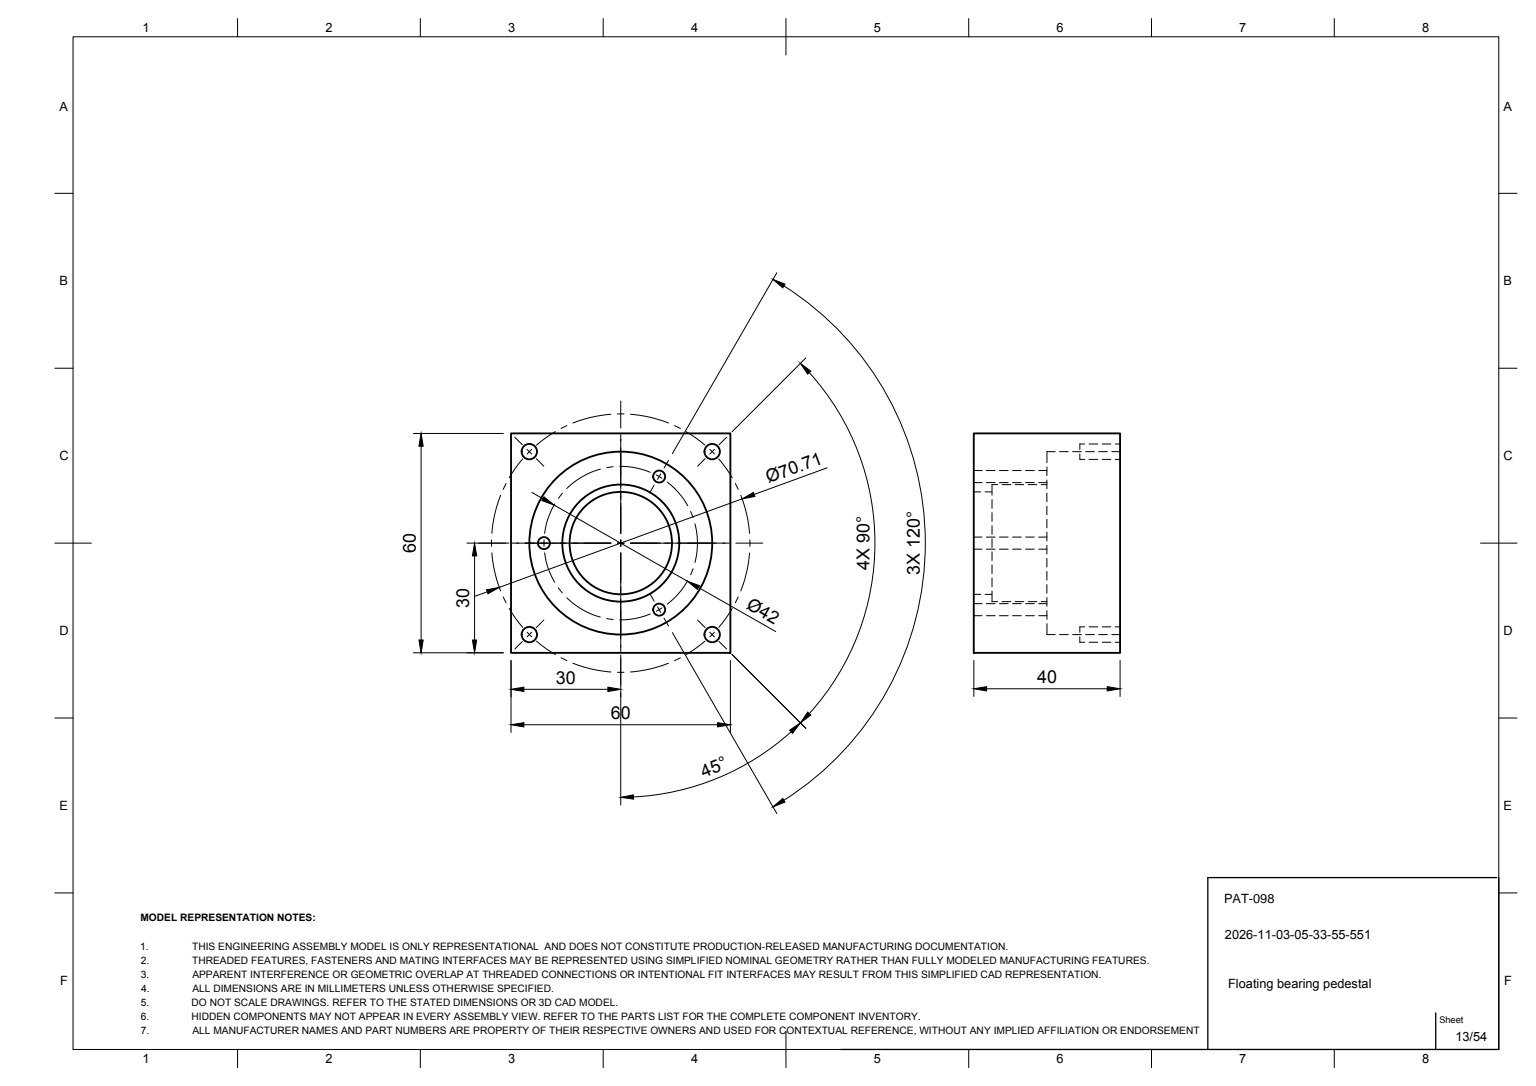
ISO-10303-21;
HEADER;
/* Generated by software containing ST-Developer
 * from STEP Tools, Inc. (www.steptools.com) 
 */

FILE_DESCRIPTION(
/* description */ ('Spring compression tester'),
/* implementation_level */ '2;1');

FILE_NAME(
/* name */ 'Floating bearing pedestal.step',
/* time_stamp */ '2026-10-28T03:24:11-07:00',
/* author */ (''),
/* organization */ (''),
/* preprocessor_version */ 'ST-DEVELOPER v20.2',
/* originating_system */ 'Autodesk Translation Framework v15.17.0.0',
/* authorisation */ '');

FILE_SCHEMA (('AUTOMOTIVE_DESIGN { 1 0 10303 214 3 1 1 }'));
ENDSEC;

DATA;
#10=MECHANICAL_DESIGN_GEOMETRIC_PRESENTATION_REPRESENTATION('',(#1114),#43521);
#994=SHAPE_REPRESENTATION_RELATIONSHIP('SRR','None',#43806,#1054);
#1054=ADVANCED_BREP_SHAPE_REPRESENTATION('',(#1189),#43466);
#1114=STYLED_ITEM('',(#44202),#1189);
#1189=MANIFOLD_SOLID_BREP('Body1',#18551);
#1345=FACE_BOUND('',#3478,.T.);
#1346=FACE_BOUND('',#3482,.T.);
#1347=FACE_BOUND('',#3483,.T.);
#1348=FACE_BOUND('',#3484,.T.);
#1349=FACE_BOUND('',#3485,.T.);
#1350=FACE_BOUND('',#3491,.T.);
#1351=FACE_BOUND('',#3492,.T.);
#1352=FACE_BOUND('',#3493,.T.);
#1353=FACE_BOUND('',#3494,.T.);
#1354=FACE_BOUND('',#3496,.T.);
#1355=FACE_BOUND('',#3497,.T.);
#1356=FACE_BOUND('',#3498,.T.);
#1357=FACE_BOUND('',#3499,.T.);
#1358=FACE_BOUND('',#3500,.T.);
#1681=PLANE('',#19583);
#1682=PLANE('',#19587);
#1683=PLANE('',#19591);
#1684=PLANE('',#19595);
#1685=PLANE('',#19599);
#1686=PLANE('',#19606);
#1687=PLANE('',#19607);
#1688=PLANE('',#19608);
#1689=PLANE('',#19609);
#1690=PLANE('',#19610);
#1691=PLANE('',#19611);
#1692=PLANE('',#19612);
#2320=FACE_OUTER_BOUND('',#3465,.T.);
#2321=FACE_OUTER_BOUND('',#3466,.T.);
#2322=FACE_OUTER_BOUND('',#3467,.T.);
#2323=FACE_OUTER_BOUND('',#3468,.T.);
#2324=FACE_OUTER_BOUND('',#3469,.T.);
#2325=FACE_OUTER_BOUND('',#3470,.T.);
#2326=FACE_OUTER_BOUND('',#3471,.T.);
#2327=FACE_OUTER_BOUND('',#3472,.T.);
#2328=FACE_OUTER_BOUND('',#3473,.T.);
#2329=FACE_OUTER_BOUND('',#3474,.T.);
#2330=FACE_OUTER_BOUND('',#3475,.T.);
#2331=FACE_OUTER_BOUND('',#3476,.T.);
#2332=FACE_OUTER_BOUND('',#3477,.T.);
#2333=FACE_OUTER_BOUND('',#3479,.T.);
#2334=FACE_OUTER_BOUND('',#3480,.T.);
#2335=FACE_OUTER_BOUND('',#3481,.T.);
#2336=FACE_OUTER_BOUND('',#3486,.T.);
#2337=FACE_OUTER_BOUND('',#3487,.T.);
#2338=FACE_OUTER_BOUND('',#3488,.T.);
#2339=FACE_OUTER_BOUND('',#3489,.T.);
#2340=FACE_OUTER_BOUND('',#3490,.T.);
#2341=FACE_OUTER_BOUND('',#3495,.T.);
#3465=EDGE_LOOP('',(#12925,#12926,#12927,#12928));
#3466=EDGE_LOOP('',(#12929,#12930,#12931,#12932));
#3467=EDGE_LOOP('',(#12933,#12934,#12935,#12936));
#3468=EDGE_LOOP('',(#12937,#12938,#12939,#12940));
#3469=EDGE_LOOP('',(#12941));
#3470=EDGE_LOOP('',(#12942,#12943,#12944,#12945));
#3471=EDGE_LOOP('',(#12946));
#3472=EDGE_LOOP('',(#12947,#12948,#12949,#12950));
#3473=EDGE_LOOP('',(#12951));
#3474=EDGE_LOOP('',(#12952,#12953,#12954,#12955));
#3475=EDGE_LOOP('',(#12956));
#3476=EDGE_LOOP('',(#12957,#12958,#12959,#12960));
#3477=EDGE_LOOP('',(#12961));
#3478=EDGE_LOOP('',(#12962));
#3479=EDGE_LOOP('',(#12963,#12964,#12965,#12966));
#3480=EDGE_LOOP('',(#12967,#12968,#12969,#12970));
#3481=EDGE_LOOP('',(#12971));
#3482=EDGE_LOOP('',(#12972));
#3483=EDGE_LOOP('',(#12973));
#3484=EDGE_LOOP('',(#12974));
#3485=EDGE_LOOP('',(#12975));
#3486=EDGE_LOOP('',(#12976,#12977,#12978,#12979));
#3487=EDGE_LOOP('',(#12980,#12981,#12982,#12983));
#3488=EDGE_LOOP('',(#12984,#12985,#12986,#12987));
#3489=EDGE_LOOP('',(#12988,#12989,#12990,#12991));
#3490=EDGE_LOOP('',(#12992,#12993,#12994,#12995));
#3491=EDGE_LOOP('',(#12996));
#3492=EDGE_LOOP('',(#12997));
#3493=EDGE_LOOP('',(#12998));
#3494=EDGE_LOOP('',(#12999));
#3495=EDGE_LOOP('',(#13000,#13001,#13002,#13003));
#3496=EDGE_LOOP('',(#13004));
#3497=EDGE_LOOP('',(#13005));
#3498=EDGE_LOOP('',(#13006));
#3499=EDGE_LOOP('',(#13007));
#3500=EDGE_LOOP('',(#13008));
#4836=LINE('',#27209,#6268);
#4837=LINE('',#27215,#6269);
#4838=LINE('',#27221,#6270);
#4839=LINE('',#27227,#6271);
#4840=LINE('',#27234,#6272);
#4841=LINE('',#27241,#6273);
#4842=LINE('',#27248,#6274);
#4843=LINE('',#27255,#6275);
#4844=LINE('',#27262,#6276);
#4845=LINE('',#27268,#6277);
#4846=LINE('',#27274,#6278);
#4847=LINE('',#27276,#6279);
#4848=LINE('',#27278,#6280);
#4849=LINE('',#27279,#6281);
#4850=LINE('',#27282,#6282);
#4851=LINE('',#27284,#6283);
#4852=LINE('',#27285,#6284);
#4853=LINE('',#27288,#6285);
#4854=LINE('',#27290,#6286);
#4855=LINE('',#27291,#6287);
#4856=LINE('',#27293,#6288);
#4857=LINE('',#27294,#6289);
#6268=VECTOR('',#22004,0.165);
#6269=VECTOR('',#22011,0.165);
#6270=VECTOR('',#22018,0.165);
#6271=VECTOR('',#22025,0.21);
#6272=VECTOR('',#22034,0.21);
#6273=VECTOR('',#22043,0.21);
#6274=VECTOR('',#22052,0.21);
#6275=VECTOR('',#22061,1.6);
#6276=VECTOR('',#22070,1.4);
#6277=VECTOR('',#22077,2.5);
#6278=VECTOR('',#22084,1.);
#6279=VECTOR('',#22085,1.);
#6280=VECTOR('',#22086,1.);
#6281=VECTOR('',#22087,1.);
#6282=VECTOR('',#22090,1.);
#6283=VECTOR('',#22091,1.);
#6284=VECTOR('',#22092,1.);
#6285=VECTOR('',#22095,1.);
#6286=VECTOR('',#22096,1.);
#6287=VECTOR('',#22097,1.);
#6288=VECTOR('',#22100,1.);
#6289=VECTOR('',#22101,1.);
#7594=CIRCLE('',#19572,0.165);
#7595=CIRCLE('',#19573,0.165);
#7596=CIRCLE('',#19575,0.165);
#7597=CIRCLE('',#19576,0.165);
#7598=CIRCLE('',#19578,0.165);
#7599=CIRCLE('',#19579,0.165);
#7600=CIRCLE('',#19581,0.21);
#7601=CIRCLE('',#19582,0.21);
#7602=CIRCLE('',#19585,0.21);
#7603=CIRCLE('',#19586,0.21);
#7604=CIRCLE('',#19589,0.21);
#7605=CIRCLE('',#19590,0.21);
#7606=CIRCLE('',#19593,0.21);
#7607=CIRCLE('',#19594,0.21);
#7608=CIRCLE('',#19597,1.6);
#7609=CIRCLE('',#19598,1.6);
#7610=CIRCLE('',#19600,1.4);
#7611=CIRCLE('',#19602,1.4);
#7612=CIRCLE('',#19604,2.5);
#7613=CIRCLE('',#19605,2.5);
#8372=VERTEX_POINT('',#27206);
#8373=VERTEX_POINT('',#27208);
#8374=VERTEX_POINT('',#27212);
#8375=VERTEX_POINT('',#27214);
#8376=VERTEX_POINT('',#27218);
#8377=VERTEX_POINT('',#27220);
#8378=VERTEX_POINT('',#27224);
#8379=VERTEX_POINT('',#27226);
#8380=VERTEX_POINT('',#27231);
#8381=VERTEX_POINT('',#27233);
#8382=VERTEX_POINT('',#27238);
#8383=VERTEX_POINT('',#27240);
#8384=VERTEX_POINT('',#27245);
#8385=VERTEX_POINT('',#27247);
#8386=VERTEX_POINT('',#27252);
#8387=VERTEX_POINT('',#27254);
#8388=VERTEX_POINT('',#27258);
#8389=VERTEX_POINT('',#27261);
#8390=VERTEX_POINT('',#27265);
#8391=VERTEX_POINT('',#27267);
#8392=VERTEX_POINT('',#27272);
#8393=VERTEX_POINT('',#27273);
#8394=VERTEX_POINT('',#27275);
#8395=VERTEX_POINT('',#27277);
#8396=VERTEX_POINT('',#27281);
#8397=VERTEX_POINT('',#27283);
#8398=VERTEX_POINT('',#27287);
#8399=VERTEX_POINT('',#27289);
#10127=EDGE_CURVE('',#8372,#8372,#7594,.T.);
#10128=EDGE_CURVE('',#8372,#8373,#4836,.T.);
#10129=EDGE_CURVE('',#8373,#8373,#7595,.T.);
#10130=EDGE_CURVE('',#8374,#8374,#7596,.T.);
#10131=EDGE_CURVE('',#8374,#8375,#4837,.T.);
#10132=EDGE_CURVE('',#8375,#8375,#7597,.T.);
#10133=EDGE_CURVE('',#8376,#8376,#7598,.T.);
#10134=EDGE_CURVE('',#8376,#8377,#4838,.T.);
#10135=EDGE_CURVE('',#8377,#8377,#7599,.T.);
#10136=EDGE_CURVE('',#8378,#8378,#7600,.T.);
#10137=EDGE_CURVE('',#8378,#8379,#4839,.T.);
#10138=EDGE_CURVE('',#8379,#8379,#7601,.T.);
#10139=EDGE_CURVE('',#8380,#8380,#7602,.T.);
#10140=EDGE_CURVE('',#8380,#8381,#4840,.T.);
#10141=EDGE_CURVE('',#8381,#8381,#7603,.T.);
#10142=EDGE_CURVE('',#8382,#8382,#7604,.T.);
#10143=EDGE_CURVE('',#8382,#8383,#4841,.T.);
#10144=EDGE_CURVE('',#8383,#8383,#7605,.T.);
#10145=EDGE_CURVE('',#8384,#8384,#7606,.T.);
#10146=EDGE_CURVE('',#8384,#8385,#4842,.T.);
#10147=EDGE_CURVE('',#8385,#8385,#7607,.T.);
#10148=EDGE_CURVE('',#8386,#8386,#7608,.T.);
#10149=EDGE_CURVE('',#8386,#8387,#4843,.T.);
#10150=EDGE_CURVE('',#8387,#8387,#7609,.T.);
#10151=EDGE_CURVE('',#8388,#8388,#7610,.T.);
#10152=EDGE_CURVE('',#8388,#8389,#4844,.T.);
#10153=EDGE_CURVE('',#8389,#8389,#7611,.T.);
#10154=EDGE_CURVE('',#8390,#8390,#7612,.T.);
#10155=EDGE_CURVE('',#8390,#8391,#4845,.T.);
#10156=EDGE_CURVE('',#8391,#8391,#7613,.T.);
#10157=EDGE_CURVE('',#8392,#8393,#4846,.T.);
#10158=EDGE_CURVE('',#8393,#8394,#4847,.T.);
#10159=EDGE_CURVE('',#8395,#8394,#4848,.T.);
#10160=EDGE_CURVE('',#8392,#8395,#4849,.T.);
#10161=EDGE_CURVE('',#8396,#8392,#4850,.T.);
#10162=EDGE_CURVE('',#8397,#8395,#4851,.T.);
#10163=EDGE_CURVE('',#8396,#8397,#4852,.T.);
#10164=EDGE_CURVE('',#8398,#8396,#4853,.T.);
#10165=EDGE_CURVE('',#8399,#8397,#4854,.T.);
#10166=EDGE_CURVE('',#8398,#8399,#4855,.T.);
#10167=EDGE_CURVE('',#8393,#8398,#4856,.T.);
#10168=EDGE_CURVE('',#8394,#8399,#4857,.T.);
#12925=ORIENTED_EDGE('',*,*,#10127,.F.);
#12926=ORIENTED_EDGE('',*,*,#10128,.T.);
#12927=ORIENTED_EDGE('',*,*,#10129,.F.);
#12928=ORIENTED_EDGE('',*,*,#10128,.F.);
#12929=ORIENTED_EDGE('',*,*,#10130,.F.);
#12930=ORIENTED_EDGE('',*,*,#10131,.T.);
#12931=ORIENTED_EDGE('',*,*,#10132,.F.);
#12932=ORIENTED_EDGE('',*,*,#10131,.F.);
#12933=ORIENTED_EDGE('',*,*,#10133,.F.);
#12934=ORIENTED_EDGE('',*,*,#10134,.T.);
#12935=ORIENTED_EDGE('',*,*,#10135,.F.);
#12936=ORIENTED_EDGE('',*,*,#10134,.F.);
#12937=ORIENTED_EDGE('',*,*,#10136,.F.);
#12938=ORIENTED_EDGE('',*,*,#10137,.T.);
#12939=ORIENTED_EDGE('',*,*,#10138,.T.);
#12940=ORIENTED_EDGE('',*,*,#10137,.F.);
#12941=ORIENTED_EDGE('',*,*,#10138,.F.);
#12942=ORIENTED_EDGE('',*,*,#10139,.F.);
#12943=ORIENTED_EDGE('',*,*,#10140,.T.);
#12944=ORIENTED_EDGE('',*,*,#10141,.T.);
#12945=ORIENTED_EDGE('',*,*,#10140,.F.);
#12946=ORIENTED_EDGE('',*,*,#10141,.F.);
#12947=ORIENTED_EDGE('',*,*,#10142,.F.);
#12948=ORIENTED_EDGE('',*,*,#10143,.T.);
#12949=ORIENTED_EDGE('',*,*,#10144,.T.);
#12950=ORIENTED_EDGE('',*,*,#10143,.F.);
#12951=ORIENTED_EDGE('',*,*,#10144,.F.);
#12952=ORIENTED_EDGE('',*,*,#10145,.F.);
#12953=ORIENTED_EDGE('',*,*,#10146,.T.);
#12954=ORIENTED_EDGE('',*,*,#10147,.T.);
#12955=ORIENTED_EDGE('',*,*,#10146,.F.);
#12956=ORIENTED_EDGE('',*,*,#10147,.F.);
#12957=ORIENTED_EDGE('',*,*,#10148,.F.);
#12958=ORIENTED_EDGE('',*,*,#10149,.T.);
#12959=ORIENTED_EDGE('',*,*,#10150,.T.);
#12960=ORIENTED_EDGE('',*,*,#10149,.F.);
#12961=ORIENTED_EDGE('',*,*,#10150,.F.);
#12962=ORIENTED_EDGE('',*,*,#10151,.F.);
#12963=ORIENTED_EDGE('',*,*,#10151,.T.);
#12964=ORIENTED_EDGE('',*,*,#10152,.T.);
#12965=ORIENTED_EDGE('',*,*,#10153,.F.);
#12966=ORIENTED_EDGE('',*,*,#10152,.F.);
#12967=ORIENTED_EDGE('',*,*,#10154,.F.);
#12968=ORIENTED_EDGE('',*,*,#10155,.T.);
#12969=ORIENTED_EDGE('',*,*,#10156,.T.);
#12970=ORIENTED_EDGE('',*,*,#10155,.F.);
#12971=ORIENTED_EDGE('',*,*,#10156,.F.);
#12972=ORIENTED_EDGE('',*,*,#10127,.T.);
#12973=ORIENTED_EDGE('',*,*,#10130,.T.);
#12974=ORIENTED_EDGE('',*,*,#10133,.T.);
#12975=ORIENTED_EDGE('',*,*,#10148,.T.);
#12976=ORIENTED_EDGE('',*,*,#10157,.T.);
#12977=ORIENTED_EDGE('',*,*,#10158,.T.);
#12978=ORIENTED_EDGE('',*,*,#10159,.F.);
#12979=ORIENTED_EDGE('',*,*,#10160,.F.);
#12980=ORIENTED_EDGE('',*,*,#10161,.T.);
#12981=ORIENTED_EDGE('',*,*,#10160,.T.);
#12982=ORIENTED_EDGE('',*,*,#10162,.F.);
#12983=ORIENTED_EDGE('',*,*,#10163,.F.);
#12984=ORIENTED_EDGE('',*,*,#10164,.T.);
#12985=ORIENTED_EDGE('',*,*,#10163,.T.);
#12986=ORIENTED_EDGE('',*,*,#10165,.F.);
#12987=ORIENTED_EDGE('',*,*,#10166,.F.);
#12988=ORIENTED_EDGE('',*,*,#10167,.T.);
#12989=ORIENTED_EDGE('',*,*,#10166,.T.);
#12990=ORIENTED_EDGE('',*,*,#10168,.F.);
#12991=ORIENTED_EDGE('',*,*,#10158,.F.);
#12992=ORIENTED_EDGE('',*,*,#10168,.T.);
#12993=ORIENTED_EDGE('',*,*,#10165,.T.);
#12994=ORIENTED_EDGE('',*,*,#10162,.T.);
#12995=ORIENTED_EDGE('',*,*,#10159,.T.);
#12996=ORIENTED_EDGE('',*,*,#10129,.T.);
#12997=ORIENTED_EDGE('',*,*,#10132,.T.);
#12998=ORIENTED_EDGE('',*,*,#10135,.T.);
#12999=ORIENTED_EDGE('',*,*,#10153,.T.);
#13000=ORIENTED_EDGE('',*,*,#10167,.F.);
#13001=ORIENTED_EDGE('',*,*,#10157,.F.);
#13002=ORIENTED_EDGE('',*,*,#10161,.F.);
#13003=ORIENTED_EDGE('',*,*,#10164,.F.);
#13004=ORIENTED_EDGE('',*,*,#10154,.T.);
#13005=ORIENTED_EDGE('',*,*,#10145,.T.);
#13006=ORIENTED_EDGE('',*,*,#10142,.T.);
#13007=ORIENTED_EDGE('',*,*,#10139,.T.);
#13008=ORIENTED_EDGE('',*,*,#10136,.T.);
#17163=CYLINDRICAL_SURFACE('',#19571,0.165);
#17164=CYLINDRICAL_SURFACE('',#19574,0.165);
#17165=CYLINDRICAL_SURFACE('',#19577,0.165);
#17166=CYLINDRICAL_SURFACE('',#19580,0.21);
#17167=CYLINDRICAL_SURFACE('',#19584,0.21);
#17168=CYLINDRICAL_SURFACE('',#19588,0.21);
#17169=CYLINDRICAL_SURFACE('',#19592,0.21);
#17170=CYLINDRICAL_SURFACE('',#19596,1.6);
#17171=CYLINDRICAL_SURFACE('',#19601,1.4);
#17172=CYLINDRICAL_SURFACE('',#19603,2.5);
#17644=ADVANCED_FACE('',(#2320),#17163,.F.);
#17645=ADVANCED_FACE('',(#2321),#17164,.F.);
#17646=ADVANCED_FACE('',(#2322),#17165,.F.);
#17647=ADVANCED_FACE('',(#2323),#17166,.F.);
#17648=ADVANCED_FACE('',(#2324),#1681,.F.);
#17649=ADVANCED_FACE('',(#2325),#17167,.F.);
#17650=ADVANCED_FACE('',(#2326),#1682,.F.);
#17651=ADVANCED_FACE('',(#2327),#17168,.F.);
#17652=ADVANCED_FACE('',(#2328),#1683,.F.);
#17653=ADVANCED_FACE('',(#2329),#17169,.F.);
#17654=ADVANCED_FACE('',(#2330),#1684,.F.);
#17655=ADVANCED_FACE('',(#2331),#17170,.F.);
#17656=ADVANCED_FACE('',(#2332,#1345),#1685,.F.);
#17657=ADVANCED_FACE('',(#2333),#17171,.F.);
#17658=ADVANCED_FACE('',(#2334),#17172,.F.);
#17659=ADVANCED_FACE('',(#2335,#1346,#1347,#1348,#1349),#1686,.F.);
#17660=ADVANCED_FACE('',(#2336),#1687,.T.);
#17661=ADVANCED_FACE('',(#2337),#1688,.T.);
#17662=ADVANCED_FACE('',(#2338),#1689,.T.);
#17663=ADVANCED_FACE('',(#2339),#1690,.T.);
#17664=ADVANCED_FACE('',(#2340,#1350,#1351,#1352,#1353),#1691,.T.);
#17665=ADVANCED_FACE('',(#2341,#1354,#1355,#1356,#1357,#1358),#1692,.F.);
#18551=CLOSED_SHELL('',(#17644,#17645,#17646,#17647,#17648,#17649,#17650,
#17651,#17652,#17653,#17654,#17655,#17656,#17657,#17658,#17659,#17660,#17661,
#17662,#17663,#17664,#17665));
#19570=AXIS2_PLACEMENT_3D('',#27204,#21998,#21999);
#19571=AXIS2_PLACEMENT_3D('',#27205,#22000,#22001);
#19572=AXIS2_PLACEMENT_3D('',#27207,#22002,#22003);
#19573=AXIS2_PLACEMENT_3D('',#27210,#22005,#22006);
#19574=AXIS2_PLACEMENT_3D('',#27211,#22007,#22008);
#19575=AXIS2_PLACEMENT_3D('',#27213,#22009,#22010);
#19576=AXIS2_PLACEMENT_3D('',#27216,#22012,#22013);
#19577=AXIS2_PLACEMENT_3D('',#27217,#22014,#22015);
#19578=AXIS2_PLACEMENT_3D('',#27219,#22016,#22017);
#19579=AXIS2_PLACEMENT_3D('',#27222,#22019,#22020);
#19580=AXIS2_PLACEMENT_3D('',#27223,#22021,#22022);
#19581=AXIS2_PLACEMENT_3D('',#27225,#22023,#22024);
#19582=AXIS2_PLACEMENT_3D('',#27228,#22026,#22027);
#19583=AXIS2_PLACEMENT_3D('',#27229,#22028,#22029);
#19584=AXIS2_PLACEMENT_3D('',#27230,#22030,#22031);
#19585=AXIS2_PLACEMENT_3D('',#27232,#22032,#22033);
#19586=AXIS2_PLACEMENT_3D('',#27235,#22035,#22036);
#19587=AXIS2_PLACEMENT_3D('',#27236,#22037,#22038);
#19588=AXIS2_PLACEMENT_3D('',#27237,#22039,#22040);
#19589=AXIS2_PLACEMENT_3D('',#27239,#22041,#22042);
#19590=AXIS2_PLACEMENT_3D('',#27242,#22044,#22045);
#19591=AXIS2_PLACEMENT_3D('',#27243,#22046,#22047);
#19592=AXIS2_PLACEMENT_3D('',#27244,#22048,#22049);
#19593=AXIS2_PLACEMENT_3D('',#27246,#22050,#22051);
#19594=AXIS2_PLACEMENT_3D('',#27249,#22053,#22054);
#19595=AXIS2_PLACEMENT_3D('',#27250,#22055,#22056);
#19596=AXIS2_PLACEMENT_3D('',#27251,#22057,#22058);
#19597=AXIS2_PLACEMENT_3D('',#27253,#22059,#22060);
#19598=AXIS2_PLACEMENT_3D('',#27256,#22062,#22063);
#19599=AXIS2_PLACEMENT_3D('',#27257,#22064,#22065);
#19600=AXIS2_PLACEMENT_3D('',#27259,#22066,#22067);
#19601=AXIS2_PLACEMENT_3D('',#27260,#22068,#22069);
#19602=AXIS2_PLACEMENT_3D('',#27263,#22071,#22072);
#19603=AXIS2_PLACEMENT_3D('',#27264,#22073,#22074);
#19604=AXIS2_PLACEMENT_3D('',#27266,#22075,#22076);
#19605=AXIS2_PLACEMENT_3D('',#27269,#22078,#22079);
#19606=AXIS2_PLACEMENT_3D('',#27270,#22080,#22081);
#19607=AXIS2_PLACEMENT_3D('',#27271,#22082,#22083);
#19608=AXIS2_PLACEMENT_3D('',#27280,#22088,#22089);
#19609=AXIS2_PLACEMENT_3D('',#27286,#22093,#22094);
#19610=AXIS2_PLACEMENT_3D('',#27292,#22098,#22099);
#19611=AXIS2_PLACEMENT_3D('',#27295,#22102,#22103);
#19612=AXIS2_PLACEMENT_3D('',#27296,#22104,#22105);
#21998=DIRECTION('axis',(0.,0.,1.));
#21999=DIRECTION('refdir',(1.,0.,0.));
#22000=DIRECTION('center_axis',(0.,0.,1.));
#22001=DIRECTION('ref_axis',(1.,0.,0.));
#22002=DIRECTION('center_axis',(0.,0.,1.));
#22003=DIRECTION('ref_axis',(1.,0.,0.));
#22004=DIRECTION('',(0.,0.,1.));
#22005=DIRECTION('center_axis',(0.,0.,-1.));
#22006=DIRECTION('ref_axis',(1.,0.,0.));
#22007=DIRECTION('center_axis',(0.,0.,1.));
#22008=DIRECTION('ref_axis',(1.,0.,0.));
#22009=DIRECTION('center_axis',(0.,0.,1.));
#22010=DIRECTION('ref_axis',(1.,0.,0.));
#22011=DIRECTION('',(0.,0.,1.));
#22012=DIRECTION('center_axis',(0.,0.,-1.));
#22013=DIRECTION('ref_axis',(1.,0.,0.));
#22014=DIRECTION('center_axis',(0.,0.,1.));
#22015=DIRECTION('ref_axis',(1.,0.,0.));
#22016=DIRECTION('center_axis',(0.,0.,1.));
#22017=DIRECTION('ref_axis',(1.,0.,0.));
#22018=DIRECTION('',(0.,0.,1.));
#22019=DIRECTION('center_axis',(0.,0.,-1.));
#22020=DIRECTION('ref_axis',(1.,0.,0.));
#22021=DIRECTION('center_axis',(0.,0.,1.));
#22022=DIRECTION('ref_axis',(1.,0.,0.));
#22023=DIRECTION('center_axis',(0.,0.,1.));
#22024=DIRECTION('ref_axis',(1.,0.,0.));
#22025=DIRECTION('',(0.,0.,1.));
#22026=DIRECTION('center_axis',(0.,0.,1.));
#22027=DIRECTION('ref_axis',(1.,0.,0.));
#22028=DIRECTION('center_axis',(0.,0.,1.));
#22029=DIRECTION('ref_axis',(1.,0.,0.));
#22030=DIRECTION('center_axis',(0.,0.,1.));
#22031=DIRECTION('ref_axis',(1.,0.,0.));
#22032=DIRECTION('center_axis',(0.,0.,1.));
#22033=DIRECTION('ref_axis',(1.,0.,0.));
#22034=DIRECTION('',(0.,0.,1.));
#22035=DIRECTION('center_axis',(0.,0.,1.));
#22036=DIRECTION('ref_axis',(1.,0.,0.));
#22037=DIRECTION('center_axis',(0.,0.,1.));
#22038=DIRECTION('ref_axis',(1.,0.,0.));
#22039=DIRECTION('center_axis',(0.,0.,1.));
#22040=DIRECTION('ref_axis',(1.,0.,0.));
#22041=DIRECTION('center_axis',(0.,0.,1.));
#22042=DIRECTION('ref_axis',(1.,0.,0.));
#22043=DIRECTION('',(0.,0.,1.));
#22044=DIRECTION('center_axis',(0.,0.,1.));
#22045=DIRECTION('ref_axis',(1.,0.,0.));
#22046=DIRECTION('center_axis',(0.,0.,1.));
#22047=DIRECTION('ref_axis',(1.,0.,0.));
#22048=DIRECTION('center_axis',(0.,0.,1.));
#22049=DIRECTION('ref_axis',(1.,0.,0.));
#22050=DIRECTION('center_axis',(0.,0.,1.));
#22051=DIRECTION('ref_axis',(1.,0.,0.));
#22052=DIRECTION('',(0.,0.,1.));
#22053=DIRECTION('center_axis',(0.,0.,1.));
#22054=DIRECTION('ref_axis',(1.,0.,0.));
#22055=DIRECTION('center_axis',(0.,0.,1.));
#22056=DIRECTION('ref_axis',(1.,0.,0.));
#22057=DIRECTION('center_axis',(0.,0.,1.));
#22058=DIRECTION('ref_axis',(1.,0.,0.));
#22059=DIRECTION('center_axis',(0.,0.,1.));
#22060=DIRECTION('ref_axis',(1.,0.,0.));
#22061=DIRECTION('',(0.,0.,1.));
#22062=DIRECTION('center_axis',(0.,0.,1.));
#22063=DIRECTION('ref_axis',(1.,0.,0.));
#22064=DIRECTION('center_axis',(0.,0.,1.));
#22065=DIRECTION('ref_axis',(1.,0.,0.));
#22066=DIRECTION('center_axis',(0.,0.,-1.));
#22067=DIRECTION('ref_axis',(1.,0.,0.));
#22068=DIRECTION('center_axis',(0.,0.,1.));
#22069=DIRECTION('ref_axis',(1.,0.,0.));
#22070=DIRECTION('',(0.,0.,1.));
#22071=DIRECTION('center_axis',(0.,0.,-1.));
#22072=DIRECTION('ref_axis',(1.,0.,0.));
#22073=DIRECTION('center_axis',(0.,0.,1.));
#22074=DIRECTION('ref_axis',(1.,0.,0.));
#22075=DIRECTION('center_axis',(0.,0.,1.));
#22076=DIRECTION('ref_axis',(1.,0.,0.));
#22077=DIRECTION('',(0.,0.,1.));
#22078=DIRECTION('center_axis',(0.,0.,1.));
#22079=DIRECTION('ref_axis',(1.,0.,0.));
#22080=DIRECTION('center_axis',(0.,0.,1.));
#22081=DIRECTION('ref_axis',(1.,0.,0.));
#22082=DIRECTION('center_axis',(0.,1.,0.));
#22083=DIRECTION('ref_axis',(-1.,0.,0.));
#22084=DIRECTION('',(-1.,0.,0.));
#22085=DIRECTION('',(0.,0.,1.));
#22086=DIRECTION('',(-1.,0.,0.));
#22087=DIRECTION('',(0.,0.,1.));
#22088=DIRECTION('center_axis',(1.,0.,0.));
#22089=DIRECTION('ref_axis',(0.,1.,0.));
#22090=DIRECTION('',(0.,1.,0.));
#22091=DIRECTION('',(0.,1.,0.));
#22092=DIRECTION('',(0.,0.,1.));
#22093=DIRECTION('center_axis',(0.,-1.,0.));
#22094=DIRECTION('ref_axis',(1.,0.,0.));
#22095=DIRECTION('',(1.,0.,0.));
#22096=DIRECTION('',(1.,0.,0.));
#22097=DIRECTION('',(0.,0.,1.));
#22098=DIRECTION('center_axis',(-1.,0.,0.));
#22099=DIRECTION('ref_axis',(0.,-1.,0.));
#22100=DIRECTION('',(0.,-1.,0.));
#22101=DIRECTION('',(0.,-1.,0.));
#22102=DIRECTION('center_axis',(0.,0.,1.));
#22103=DIRECTION('ref_axis',(1.,0.,0.));
#22104=DIRECTION('center_axis',(0.,0.,1.));
#22105=DIRECTION('ref_axis',(1.,0.,0.));
#27204=CARTESIAN_POINT('',(0.,0.,0.));
#27205=CARTESIAN_POINT('Origin',(2.1,5.,1.9));
#27206=CARTESIAN_POINT('',(1.935,5.,2.));
#27207=CARTESIAN_POINT('Origin',(2.1,5.,2.));
#27208=CARTESIAN_POINT('',(1.935,5.,4.));
#27209=CARTESIAN_POINT('',(1.935,5.,1.9));
#27210=CARTESIAN_POINT('Origin',(2.1,5.,4.));
#27211=CARTESIAN_POINT('Origin',(-1.05,6.81865334794732,1.9));
#27212=CARTESIAN_POINT('',(-1.215,6.81865334794732,2.));
#27213=CARTESIAN_POINT('Origin',(-1.05,6.81865334794732,2.));
#27214=CARTESIAN_POINT('',(-1.215,6.81865334794732,4.));
#27215=CARTESIAN_POINT('',(-1.215,6.81865334794732,1.9));
#27216=CARTESIAN_POINT('Origin',(-1.05,6.81865334794732,4.));
#27217=CARTESIAN_POINT('Origin',(-1.05,3.18134665205268,1.9));
#27218=CARTESIAN_POINT('',(-1.215,3.18134665205268,2.));
#27219=CARTESIAN_POINT('Origin',(-1.05,3.18134665205268,2.));
#27220=CARTESIAN_POINT('',(-1.215,3.18134665205268,4.));
#27221=CARTESIAN_POINT('',(-1.215,3.18134665205268,1.9));
#27222=CARTESIAN_POINT('Origin',(-1.05,3.18134665205268,4.));
#27223=CARTESIAN_POINT('Origin',(2.5,2.5,-0.1));
#27224=CARTESIAN_POINT('',(2.29,2.5,0.));
#27225=CARTESIAN_POINT('Origin',(2.5,2.5,0.));
#27226=CARTESIAN_POINT('',(2.29,2.5,1.1));
#27227=CARTESIAN_POINT('',(2.29,2.5,-0.1));
#27228=CARTESIAN_POINT('Origin',(2.5,2.5,1.1));
#27229=CARTESIAN_POINT('Origin',(2.5,2.5,1.1));
#27230=CARTESIAN_POINT('Origin',(-2.5,7.5,-0.1));
#27231=CARTESIAN_POINT('',(-2.71,7.5,0.));
#27232=CARTESIAN_POINT('Origin',(-2.5,7.5,0.));
#27233=CARTESIAN_POINT('',(-2.71,7.5,1.1));
#27234=CARTESIAN_POINT('',(-2.71,7.5,-0.1));
#27235=CARTESIAN_POINT('Origin',(-2.5,7.5,1.1));
#27236=CARTESIAN_POINT('Origin',(-2.5,7.5,1.1));
#27237=CARTESIAN_POINT('Origin',(-2.5,2.5,-0.1));
#27238=CARTESIAN_POINT('',(-2.71,2.5,0.));
#27239=CARTESIAN_POINT('Origin',(-2.5,2.5,0.));
#27240=CARTESIAN_POINT('',(-2.71,2.5,1.1));
#27241=CARTESIAN_POINT('',(-2.71,2.5,-0.1));
#27242=CARTESIAN_POINT('Origin',(-2.5,2.5,1.1));
#27243=CARTESIAN_POINT('Origin',(-2.5,2.5,1.1));
#27244=CARTESIAN_POINT('Origin',(2.5,7.5,-0.1));
#27245=CARTESIAN_POINT('',(2.29,7.5,0.));
#27246=CARTESIAN_POINT('Origin',(2.5,7.5,0.));
#27247=CARTESIAN_POINT('',(2.29,7.5,1.1));
#27248=CARTESIAN_POINT('',(2.29,7.5,-0.1));
#27249=CARTESIAN_POINT('Origin',(2.5,7.5,1.1));
#27250=CARTESIAN_POINT('Origin',(2.5,7.5,1.1));
#27251=CARTESIAN_POINT('Origin',(0.,5.,1.9));
#27252=CARTESIAN_POINT('',(-1.6,5.,2.));
#27253=CARTESIAN_POINT('Origin',(0.,5.,2.));
#27254=CARTESIAN_POINT('',(-1.6,5.,3.5));
#27255=CARTESIAN_POINT('',(-1.6,5.,1.9));
#27256=CARTESIAN_POINT('Origin',(0.,5.,3.5));
#27257=CARTESIAN_POINT('Origin',(0.,5.,3.5));
#27258=CARTESIAN_POINT('',(-1.4,5.,3.5));
#27259=CARTESIAN_POINT('Origin',(0.,5.,3.5));
#27260=CARTESIAN_POINT('Origin',(0.,5.,1.9));
#27261=CARTESIAN_POINT('',(-1.4,5.,4.));
#27262=CARTESIAN_POINT('',(-1.4,5.,1.9));
#27263=CARTESIAN_POINT('Origin',(0.,5.,4.));
#27264=CARTESIAN_POINT('Origin',(0.,5.,-0.1));
#27265=CARTESIAN_POINT('',(-2.5,5.,0.));
#27266=CARTESIAN_POINT('Origin',(0.,5.,0.));
#27267=CARTESIAN_POINT('',(-2.5,5.,2.));
#27268=CARTESIAN_POINT('',(-2.5,5.,-0.1));
#27269=CARTESIAN_POINT('Origin',(0.,5.,2.));
#27270=CARTESIAN_POINT('Origin',(0.,5.,2.));
#27271=CARTESIAN_POINT('Origin',(3.,8.,0.));
#27272=CARTESIAN_POINT('',(3.,8.,0.));
#27273=CARTESIAN_POINT('',(-3.,8.,0.));
#27274=CARTESIAN_POINT('',(3.,8.,0.));
#27275=CARTESIAN_POINT('',(-3.,8.,4.));
#27276=CARTESIAN_POINT('',(-3.,8.,0.));
#27277=CARTESIAN_POINT('',(3.,8.,4.));
#27278=CARTESIAN_POINT('',(3.,8.,4.));
#27279=CARTESIAN_POINT('',(3.,8.,0.));
#27280=CARTESIAN_POINT('Origin',(3.,2.,0.));
#27281=CARTESIAN_POINT('',(3.,2.,0.));
#27282=CARTESIAN_POINT('',(3.,2.,0.));
#27283=CARTESIAN_POINT('',(3.,2.,4.));
#27284=CARTESIAN_POINT('',(3.,2.,4.));
#27285=CARTESIAN_POINT('',(3.,2.,0.));
#27286=CARTESIAN_POINT('Origin',(-3.,2.,0.));
#27287=CARTESIAN_POINT('',(-3.,2.,0.));
#27288=CARTESIAN_POINT('',(-3.,2.,0.));
#27289=CARTESIAN_POINT('',(-3.,2.,4.));
#27290=CARTESIAN_POINT('',(-3.,2.,4.));
#27291=CARTESIAN_POINT('',(-3.,2.,0.));
#27292=CARTESIAN_POINT('Origin',(-3.,8.,0.));
#27293=CARTESIAN_POINT('',(-3.,8.,0.));
#27294=CARTESIAN_POINT('',(-3.,8.,4.));
#27295=CARTESIAN_POINT('Origin',(0.,5.,4.));
#27296=CARTESIAN_POINT('Origin',(0.,5.,0.));
#43398=UNCERTAINTY_MEASURE_WITH_UNIT(LENGTH_MEASURE(0.001),#43522,
'DISTANCE_ACCURACY_VALUE',
'Maximum model space distance between geometric entities at asserted c
onnectivities');
#43453=UNCERTAINTY_MEASURE_WITH_UNIT(LENGTH_MEASURE(0.001),#43522,
'DISTANCE_ACCURACY_VALUE',
'Maximum model space distance between geometric entities at asserted c
onnectivities');
#43466=(
GEOMETRIC_REPRESENTATION_CONTEXT(3)
GLOBAL_UNCERTAINTY_ASSIGNED_CONTEXT((#43398))
GLOBAL_UNIT_ASSIGNED_CONTEXT((#43522,#43524,#43525))
REPRESENTATION_CONTEXT('','3D')
);
#43521=(
GEOMETRIC_REPRESENTATION_CONTEXT(3)
GLOBAL_UNCERTAINTY_ASSIGNED_CONTEXT((#43453))
GLOBAL_UNIT_ASSIGNED_CONTEXT((#43522,#43524,#43525))
REPRESENTATION_CONTEXT('','3D')
);
#43522=(
LENGTH_UNIT()
NAMED_UNIT(*)
SI_UNIT(.CENTI.,.METRE.)
);
#43524=(
NAMED_UNIT(*)
PLANE_ANGLE_UNIT()
SI_UNIT($,.RADIAN.)
);
#43525=(
NAMED_UNIT(*)
SI_UNIT($,.STERADIAN.)
SOLID_ANGLE_UNIT()
);
#43538=SHAPE_DEFINITION_REPRESENTATION(#43605,#43806);
#43605=PRODUCT_DEFINITION_SHAPE('',$,#43874);
#43806=SHAPE_REPRESENTATION('',(#19570),#43466);
#43861=PRODUCT_DEFINITION_CONTEXT('part definition',#44064,'design');
#43874=PRODUCT_DEFINITION('Floating bearing pedestal',
'Floating bearing pedestal',#43941,#43861);
#43941=PRODUCT_DEFINITION_FORMATION('',$,#44078);
#44064=APPLICATION_CONTEXT(
'Core Data for Automotive Mechanical Design Process');
#44065=PRODUCT_CONTEXT('part definition',#44064,'mechanical');
#44078=PRODUCT('Floating bearing pedestal','Floating bearing pedestal',
'Floating bearing pedestal',(#44065));
#44196=COLOUR_RGB('Grey',0.48,0.52,0.57);
#44197=FILL_AREA_STYLE_COLOUR('',#44196);
#44198=FILL_AREA_STYLE('',(#44197));
#44199=SURFACE_STYLE_FILL_AREA(#44198);
#44200=SURFACE_SIDE_STYLE('',(#44199));
#44201=SURFACE_STYLE_USAGE(.BOTH.,#44200);
#44202=PRESENTATION_STYLE_ASSIGNMENT((#44201));
ENDSEC;
END-ISO-10303-21;
